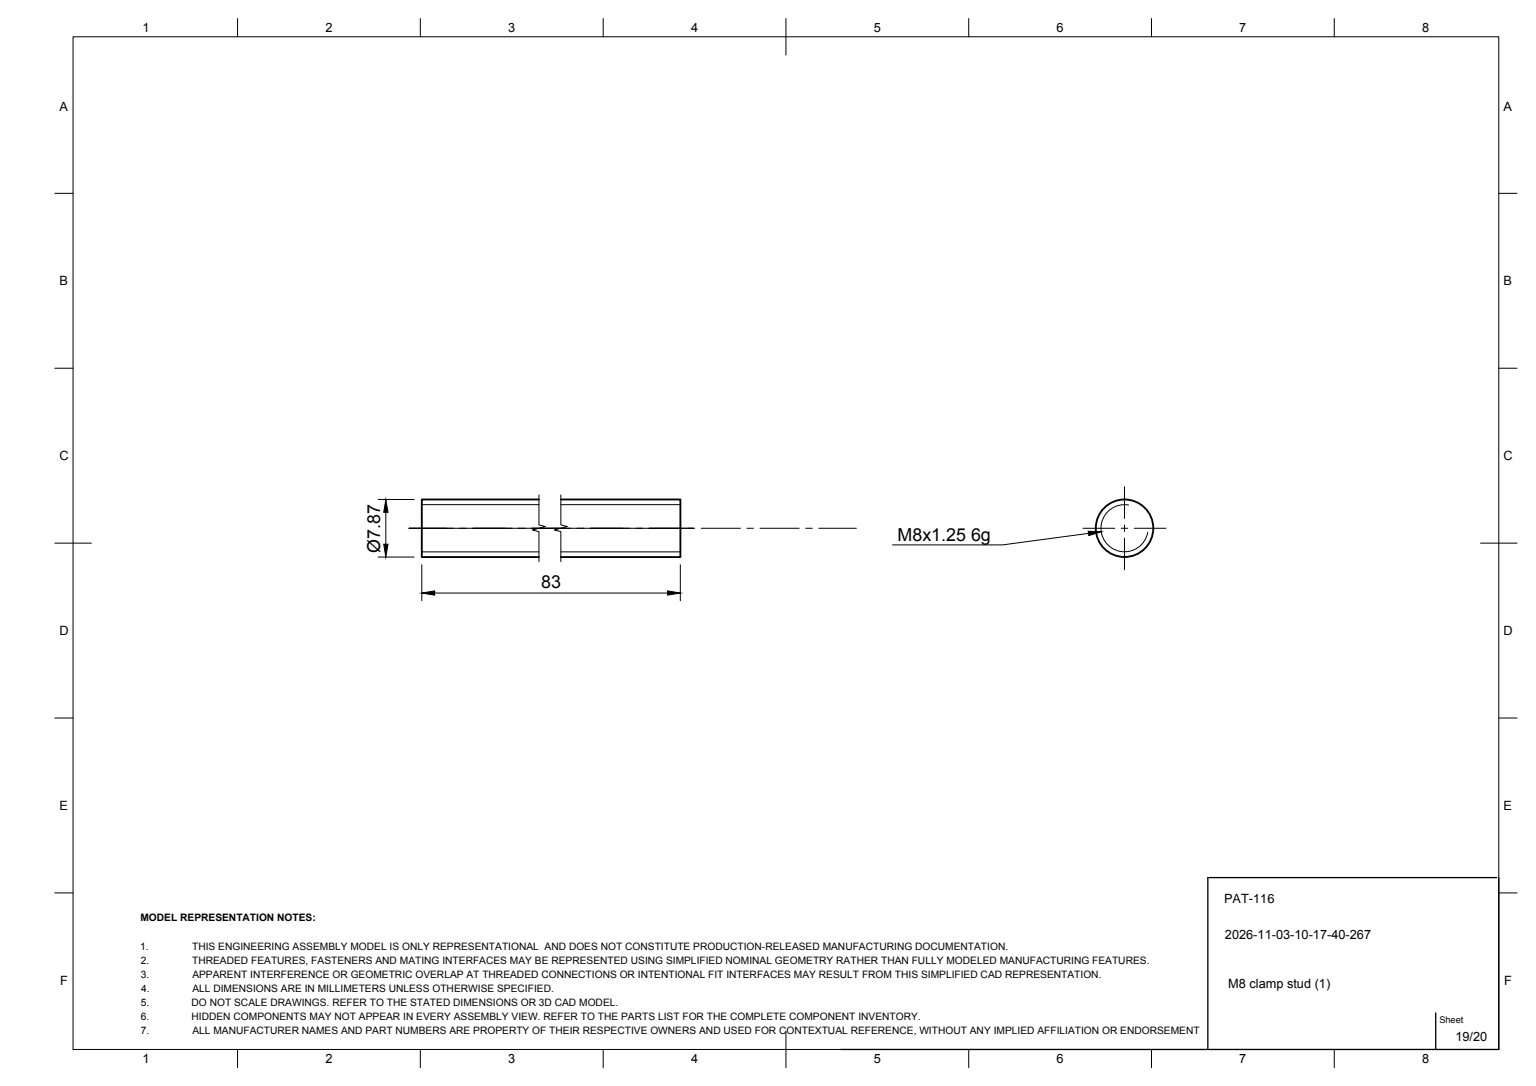
ISO-10303-21;
HEADER;
/* Generated by software containing ST-Developer
 * from STEP Tools, Inc. (www.steptools.com) 
 */

FILE_DESCRIPTION(
/* description */ ('V-block with clamp strap'),
/* implementation_level */ '2;1');

FILE_NAME(
/* name */ 'M8 clamp stud (1).step',
/* time_stamp */ '2026-10-27T10:50:53-07:00',
/* author */ (''),
/* organization */ (''),
/* preprocessor_version */ 'ST-DEVELOPER v20.2',
/* originating_system */ 'Autodesk Translation Framework v15.17.0.0',
/* authorisation */ '');

FILE_SCHEMA (('AUTOMOTIVE_DESIGN { 1 0 10303 214 3 1 1 }'));
ENDSEC;

DATA;
#10=MECHANICAL_DESIGN_GEOMETRIC_PRESENTATION_REPRESENTATION('',(#282),#7344);
#240=SHAPE_REPRESENTATION_RELATIONSHIP('SRR','None',#7459,#261);
#261=ADVANCED_BREP_SHAPE_REPRESENTATION('',(#301),#7338);
#282=STYLED_ITEM('',(#7638),#301);
#301=MANIFOLD_SOLID_BREP('Body1',#4166);
#486=CIRCLE('',#4765,0.3933);
#487=CIRCLE('',#4766,0.3933);
#555=CYLINDRICAL_SURFACE('',#4764,0.3933);
#765=FACE_OUTER_BOUND('',#1071,.T.);
#766=FACE_OUTER_BOUND('',#1072,.T.);
#767=FACE_OUTER_BOUND('',#1073,.T.);
#1071=EDGE_LOOP('',(#3606,#3607,#3608,#3609));
#1072=EDGE_LOOP('',(#3610));
#1073=EDGE_LOOP('',(#3611));
#1442=LINE('',#7103,#1807);
#1807=VECTOR('',#5896,0.4);
#2131=VERTEX_POINT('',#7100);
#2132=VERTEX_POINT('',#7102);
#2629=EDGE_CURVE('',#2131,#2131,#486,.F.);
#2630=EDGE_CURVE('',#2131,#2132,#1442,.T.);
#2631=EDGE_CURVE('',#2132,#2132,#487,.F.);
#3606=ORIENTED_EDGE('',*,*,#2629,.F.);
#3607=ORIENTED_EDGE('',*,*,#2630,.T.);
#3608=ORIENTED_EDGE('',*,*,#2631,.T.);
#3609=ORIENTED_EDGE('',*,*,#2630,.F.);
#3610=ORIENTED_EDGE('',*,*,#2629,.T.);
#3611=ORIENTED_EDGE('',*,*,#2631,.F.);
#3883=PLANE('',#4767);
#3884=PLANE('',#4768);
#4111=ADVANCED_FACE('',(#765),#555,.T.);
#4112=ADVANCED_FACE('',(#766),#3883,.T.);
#4113=ADVANCED_FACE('',(#767),#3884,.F.);
#4166=CLOSED_SHELL('',(#4111,#4112,#4113));
#4763=AXIS2_PLACEMENT_3D('',#7098,#5890,#5891);
#4764=AXIS2_PLACEMENT_3D('',#7099,#5892,#5893);
#4765=AXIS2_PLACEMENT_3D('',#7101,#5894,#5895);
#4766=AXIS2_PLACEMENT_3D('',#7104,#5897,#5898);
#4767=AXIS2_PLACEMENT_3D('',#7105,#5899,#5900);
#4768=AXIS2_PLACEMENT_3D('',#7106,#5901,#5902);
#5890=DIRECTION('axis',(0.,0.,1.));
#5891=DIRECTION('refdir',(1.,0.,0.));
#5892=DIRECTION('center_axis',(0.,0.,1.));
#5893=DIRECTION('ref_axis',(1.,0.,0.));
#5894=DIRECTION('center_axis',(0.,0.,-1.));
#5895=DIRECTION('ref_axis',(1.,0.,0.));
#5896=DIRECTION('',(0.,0.,-1.));
#5897=DIRECTION('center_axis',(0.,0.,-1.));
#5898=DIRECTION('ref_axis',(1.,0.,0.));
#5899=DIRECTION('center_axis',(0.,0.,1.));
#5900=DIRECTION('ref_axis',(1.,0.,0.));
#5901=DIRECTION('center_axis',(0.,0.,1.));
#5902=DIRECTION('ref_axis',(1.,0.,0.));
#7098=CARTESIAN_POINT('',(0.,0.,0.));
#7099=CARTESIAN_POINT('Origin',(10.,4.,0.));
#7100=CARTESIAN_POINT('',(9.6067,4.,8.3));
#7101=CARTESIAN_POINT('Origin',(10.,4.,8.3));
#7102=CARTESIAN_POINT('',(9.6067,4.,0.));
#7103=CARTESIAN_POINT('',(9.6067,4.,0.));
#7104=CARTESIAN_POINT('Origin',(10.,4.,0.));
#7105=CARTESIAN_POINT('Origin',(10.,4.,8.3));
#7106=CARTESIAN_POINT('Origin',(10.,4.,0.));
#7312=UNCERTAINTY_MEASURE_WITH_UNIT(LENGTH_MEASURE(0.001),#7345,
'DISTANCE_ACCURACY_VALUE',
'Maximum model space distance between geometric entities at asserted c
onnectivities');
#7318=UNCERTAINTY_MEASURE_WITH_UNIT(LENGTH_MEASURE(0.001),#7345,
'DISTANCE_ACCURACY_VALUE',
'Maximum model space distance between geometric entities at asserted c
onnectivities');
#7338=(
GEOMETRIC_REPRESENTATION_CONTEXT(3)
GLOBAL_UNCERTAINTY_ASSIGNED_CONTEXT((#7312))
GLOBAL_UNIT_ASSIGNED_CONTEXT((#7345,#7347,#7348))
REPRESENTATION_CONTEXT('','3D')
);
#7344=(
GEOMETRIC_REPRESENTATION_CONTEXT(3)
GLOBAL_UNCERTAINTY_ASSIGNED_CONTEXT((#7318))
GLOBAL_UNIT_ASSIGNED_CONTEXT((#7345,#7347,#7348))
REPRESENTATION_CONTEXT('','3D')
);
#7345=(
LENGTH_UNIT()
NAMED_UNIT(*)
SI_UNIT(.CENTI.,.METRE.)
);
#7347=(
NAMED_UNIT(*)
PLANE_ANGLE_UNIT()
SI_UNIT($,.RADIAN.)
);
#7348=(
NAMED_UNIT(*)
SI_UNIT($,.STERADIAN.)
SOLID_ANGLE_UNIT()
);
#7368=SHAPE_DEFINITION_REPRESENTATION(#7416,#7459);
#7416=PRODUCT_DEFINITION_SHAPE('',$,#7485);
#7459=SHAPE_REPRESENTATION('',(#4763),#7338);
#7465=PRODUCT_DEFINITION_CONTEXT('part definition',#7542,'design');
#7485=PRODUCT_DEFINITION('M8 clamp stud (1)','M8 clamp stud (1)',#7510,#7465);
#7510=PRODUCT_DEFINITION_FORMATION('',$,#7563);
#7542=APPLICATION_CONTEXT(
'Core Data for Automotive Mechanical Design Process');
#7543=PRODUCT_CONTEXT('part definition',#7542,'mechanical');
#7563=PRODUCT('M8 clamp stud (1)','M8 clamp stud (1)','M8 clamp stud (1)',(#7543));
#7632=COLOUR_RGB('Black',0.12,0.14,0.17);
#7633=FILL_AREA_STYLE_COLOUR('',#7632);
#7634=FILL_AREA_STYLE('',(#7633));
#7635=SURFACE_STYLE_FILL_AREA(#7634);
#7636=SURFACE_SIDE_STYLE('',(#7635));
#7637=SURFACE_STYLE_USAGE(.BOTH.,#7636);
#7638=PRESENTATION_STYLE_ASSIGNMENT((#7637));
ENDSEC;
END-ISO-10303-21;
